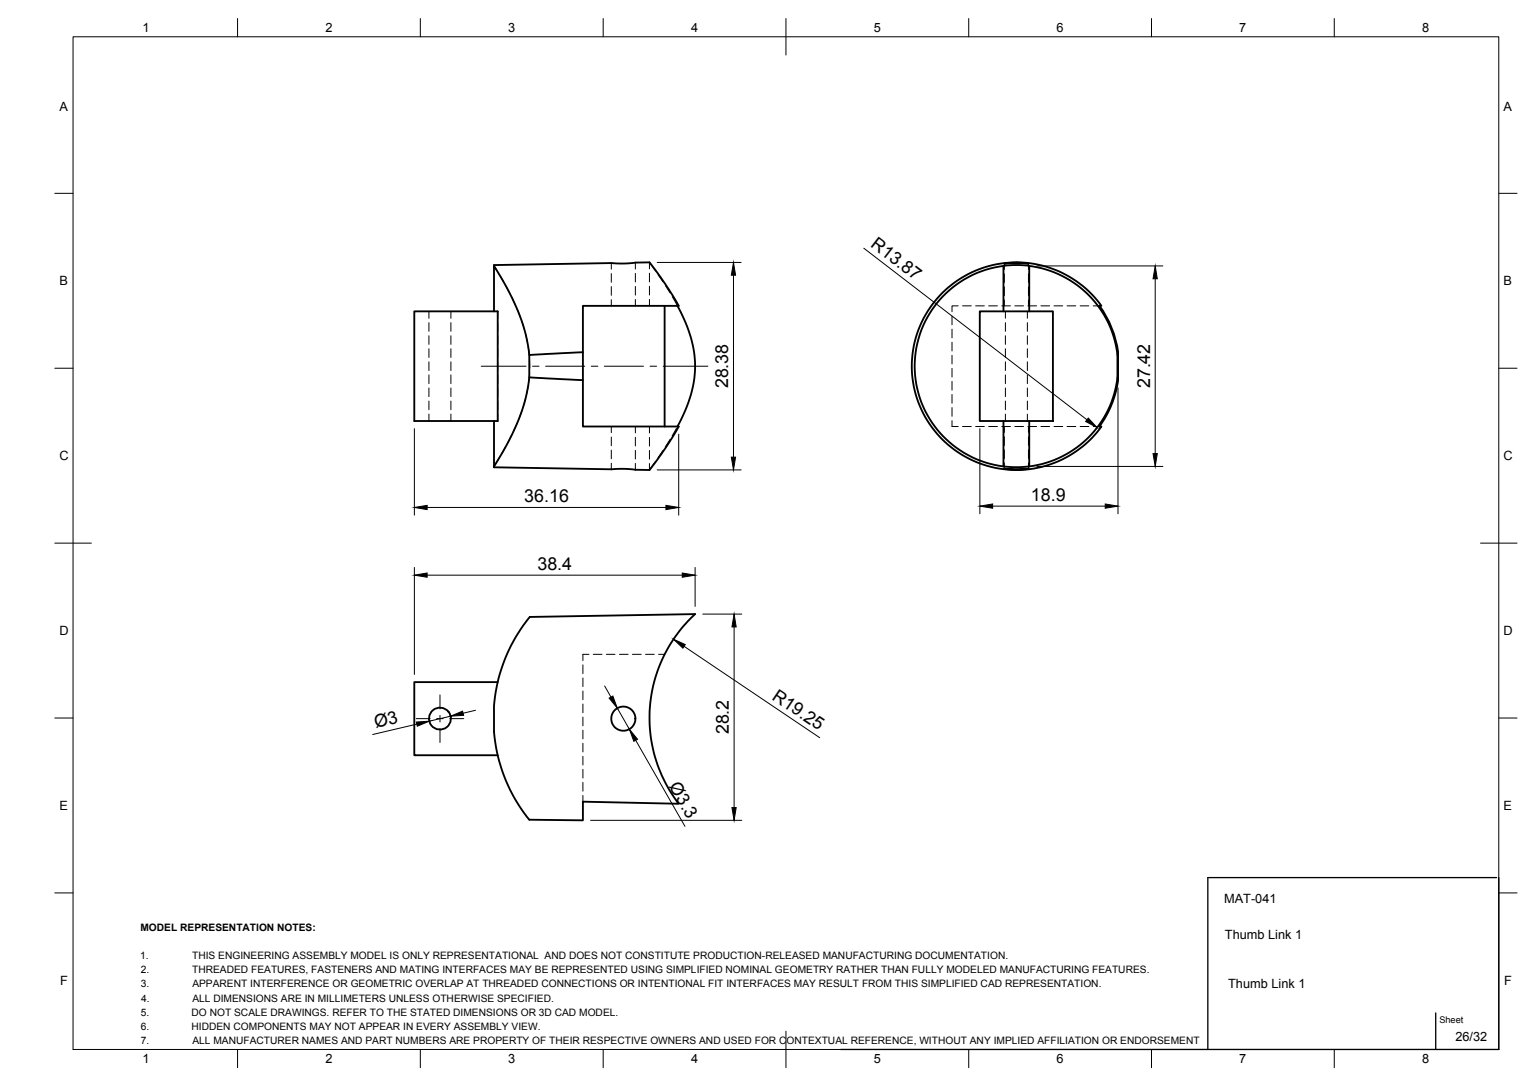
ISO-10303-21;
HEADER;
/* Generated by software containing ST-Developer
 * from STEP Tools, Inc. (www.steptools.com) 
 */

FILE_DESCRIPTION(
/* description */ ('STEP AP214'),
/* implementation_level */ '2;1');

FILE_NAME(
/* name */ 'Thumb Link 1.step',
/* time_stamp */ '2026-11-14T21:57:47-08:00',
/* author */ (''),
/* organization */ (''),
/* preprocessor_version */ 'ST-DEVELOPER v20.2',
/* originating_system */ 'Autodesk Translation Framework v15.17.0.0',
/* authorisation */ '');

FILE_SCHEMA (('AUTOMOTIVE_DESIGN { 1 0 10303 214 3 1 1 }'));
ENDSEC;

DATA;
#10=MECHANICAL_DESIGN_GEOMETRIC_PRESENTATION_REPRESENTATION('',(#261),#13199);
#12=(
BOUNDED_CURVE()
B_SPLINE_CURVE(2,(#12481,#12482,#12483),.UNSPECIFIED.,.F.,.F.)
B_SPLINE_CURVE_WITH_KNOTS((3,3),(-1.60124615225297,-0.808783730274253),
 .UNSPECIFIED.)
CURVE()
GEOMETRIC_REPRESENTATION_ITEM()
RATIONAL_B_SPLINE_CURVE((1.00284139361103,1.00297035013721,1.00227572336188))
REPRESENTATION_ITEM('')
);
#13=(
BOUNDED_CURVE()
B_SPLINE_CURVE(2,(#12547,#12548,#12549),.UNSPECIFIED.,.F.,.F.)
B_SPLINE_CURVE_WITH_KNOTS((3,3),(-2.14592066681242,-1.35342729440919),
 .UNSPECIFIED.)
CURVE()
GEOMETRIC_REPRESENTATION_ITEM()
RATIONAL_B_SPLINE_CURVE((1.00227603694351,1.00297081766941,1.00284201479666))
REPRESENTATION_ITEM('')
);
#123=CONICAL_SURFACE('',#7682,14.3,0.0174532925199433);
#189=B_SPLINE_CURVE_WITH_KNOTS('',3,(#12314,#12315,#12316,#12317,#12318,
#12319,#12320,#12321,#12322,#12323,#12324,#12325,#12326,#12327,#12328,#12329,
#12330,#12331),.UNSPECIFIED.,.F.,.F.,(4,2,2,2,2,2,2,2,4),(1.2439344005176,
1.30605868780294,1.36818297508828,1.43027366468746,1.49236435428665,1.55470347254014,
1.61704259079363,1.67936460734276,1.74168662389188),.UNSPECIFIED.);
#190=B_SPLINE_CURVE_WITH_KNOTS('',3,(#12332,#12333,#12334,#12335,#12336,
#12337,#12338,#12339,#12340,#12341,#12342,#12343,#12344,#12345,#12346,#12347,
#12348,#12349,#12350),.UNSPECIFIED.,.F.,.F.,(4,2,2,2,3,2,2,2,4),(0.746182177143323,
0.80850419369245,0.870826210241576,0.933165328495069,0.995504446748561,
1.05759513634774,1.11968582594693,1.18181011323227,1.2439344005176),
 .UNSPECIFIED.);
#191=B_SPLINE_CURVE_WITH_KNOTS('',3,(#12354,#12355,#12356,#12357,#12358,
#12359,#12360,#12361,#12362,#12363,#12364,#12365,#12366,#12367,#12368,#12369,
#12370,#12371),.UNSPECIFIED.,.F.,.F.,(4,2,2,2,2,2,2,2,4),(-0.746182177143323,
-0.683860160594197,-0.621538144045071,-0.559199025791578,-0.496859907538086,
-0.434769217938902,-0.372678528339718,-0.310554241054381,-0.248429953769043),
 .UNSPECIFIED.);
#192=B_SPLINE_CURVE_WITH_KNOTS('',3,(#12375,#12376,#12377,#12378,#12379,
#12380,#12381,#12382,#12383,#12384,#12385,#12386,#12387,#12388,#12389,#12390,
#12391,#12392,#12393),.UNSPECIFIED.,.F.,.F.,(4,2,2,2,3,2,2,2,4),(-0.248429953769043,
-0.186305666483705,-0.124181379198368,-0.0620906895991839,0.,0.0623391182534924,
0.124678236506985,0.187000253056111,0.249322269605238),.UNSPECIFIED.);
#193=B_SPLINE_CURVE_WITH_KNOTS('',3,(#12409,#12410,#12411,#12412,#12413,
#12414,#12415,#12416,#12417,#12418,#12419,#12420,#12421,#12422),
 .UNSPECIFIED.,.F.,.F.,(4,2,2,2,2,2,4),(6.66820605648738,6.76341848404012,
7.03258976532484,7.57093232789428,8.11497235847169,8.3869923737604,8.50692180294266),
 .UNSPECIFIED.);
#194=B_SPLINE_CURVE_WITH_KNOTS('',3,(#12426,#12427,#12428,#12429,#12430,
#12431,#12432,#12433,#12434,#12435,#12436,#12437,#12438,#12439),
 .UNSPECIFIED.,.F.,.F.,(4,2,2,2,2,2,4),(0.152090586106455,0.272020015288707,
0.544040030577415,1.08808006115483,1.62642262372427,1.89559390500899,1.99080633256173),
 .UNSPECIFIED.);
#195=B_SPLINE_CURVE_WITH_KNOTS('',3,(#12452,#12453,#12454,#12455,#12456,
#12457,#12458,#12459,#12460,#12461,#12462,#12463,#12464,#12465,#12466,#12467,
#12468,#12469,#12470,#12471,#12472,#12473,#12474,#12475,#12476,#12477),
 .UNSPECIFIED.,.F.,.F.,(4,2,2,2,2,2,2,2,2,2,2,2,4),(2.33883536058546,2.43393235013178,
2.70309951396985,3.24143384164599,3.78547001808527,4.05748810630491,4.32950619452455,
4.6015242827442,4.87354237096384,5.41757854740312,5.95591287507926,6.22508003891732,
6.32017702846365),.UNSPECIFIED.);
#196=B_SPLINE_CURVE_WITH_KNOTS('',3,(#12487,#12488,#12489,#12490,#12491,
#12492,#12493),.UNSPECIFIED.,.F.,.F.,(4,3,4),(0.0272601210138638,0.0280070000945348,
0.0403698029815644),.UNSPECIFIED.);
#197=B_SPLINE_CURVE_WITH_KNOTS('',3,(#12495,#12496,#12497,#12498,#12499,
#12500,#12501,#12502,#12503,#12504,#12505,#12506,#12507,#12508,#12509,#12510,
#12511,#12512,#12513,#12514,#12515,#12516,#12517,#12518,#12519,#12520,#12521,
#12522,#12523,#12524,#12525,#12526,#12527,#12528,#12529,#12530,#12531,#12532,
#12533,#12534,#12535,#12536),.UNSPECIFIED.,.F.,.F.,(4,2,2,2,2,2,2,2,2,2,
2,2,2,2,2,2,2,2,2,2,4),(0.895792364322182,1.15266269025927,1.7130326392156,
1.99321761369377,2.27340258817193,2.55312809524007,2.8328536023082,3.39230461644446,
3.9653006408784,4.25179865309537,4.53829666531233,4.8247946775293,5.11129268974627,
5.6842887141802,6.24373972831647,6.5234652353846,6.80319074245273,7.08415066001029,
7.36511057756785,7.92703041268297,8.1809357022053),.UNSPECIFIED.);
#198=B_SPLINE_CURVE_WITH_KNOTS('',3,(#12538,#12539,#12540,#12541,#12542,
#12543,#12544),.UNSPECIFIED.,.F.,.F.,(4,3,4),(0.01564419735118,0.0280070001942108,
0.0287538792722237),.UNSPECIFIED.);
#225=SHAPE_REPRESENTATION_RELATIONSHIP('SRR','None',#13297,#243);
#243=ADVANCED_BREP_SHAPE_REPRESENTATION('',(#279),#13193);
#261=STYLED_ITEM('',(#13411),#279);
#279=MANIFOLD_SOLID_BREP('Body1',#6856);
#362=FACE_BOUND('',#2584,.T.);
#363=FACE_BOUND('',#2585,.T.);
#364=FACE_BOUND('',#2590,.T.);
#365=FACE_BOUND('',#2592,.T.);
#366=FACE_BOUND('',#2599,.T.);
#367=FACE_BOUND('',#2601,.T.);
#561=PLANE('',#7674);
#562=PLANE('',#7686);
#563=PLANE('',#7687);
#564=PLANE('',#7691);
#565=PLANE('',#7692);
#566=PLANE('',#7693);
#567=PLANE('',#7694);
#568=PLANE('',#7695);
#569=PLANE('',#7696);
#570=PLANE('',#7697);
#571=PLANE('',#7698);
#572=PLANE('',#7699);
#1017=LINE('',#12306,#1535);
#1018=LINE('',#12312,#1536);
#1019=LINE('',#12373,#1537);
#1020=LINE('',#12397,#1538);
#1021=LINE('',#12399,#1539);
#1022=LINE('',#12401,#1540);
#1023=LINE('',#12406,#1541);
#1024=LINE('',#12424,#1542);
#1025=LINE('',#12441,#1543);
#1026=LINE('',#12447,#1544);
#1027=LINE('',#12451,#1545);
#1028=LINE('',#12551,#1546);
#1029=LINE('',#12553,#1547);
#1030=LINE('',#12557,#1548);
#1031=LINE('',#12562,#1549);
#1032=LINE('',#12563,#1550);
#1033=LINE('',#12566,#1551);
#1034=LINE('',#12567,#1552);
#1035=LINE('',#12569,#1553);
#1036=LINE('',#12573,#1554);
#1037=LINE('',#12575,#1555);
#1038=LINE('',#12576,#1556);
#1039=LINE('',#12579,#1557);
#1040=LINE('',#12581,#1558);
#1041=LINE('',#12582,#1559);
#1042=LINE('',#12584,#1560);
#1043=LINE('',#12585,#1561);
#1535=VECTOR('',#9454,1.5);
#1536=VECTOR('',#9461,1.65);
#1537=VECTOR('',#9464,1.65);
#1538=VECTOR('',#9469,1000.);
#1539=VECTOR('',#9470,1000.);
#1540=VECTOR('',#9471,1000.);
#1541=VECTOR('',#9476,1000.);
#1542=VECTOR('',#9479,1000.);
#1543=VECTOR('',#9480,1000.);
#1544=VECTOR('',#9487,1000.);
#1545=VECTOR('',#9490,1000.);
#1546=VECTOR('',#9501,1000.);
#1547=VECTOR('',#9504,1000.);
#1548=VECTOR('',#9507,1000.);
#1549=VECTOR('',#9514,1000.);
#1550=VECTOR('',#9515,1000.);
#1551=VECTOR('',#9518,1000.);
#1552=VECTOR('',#9519,1000.);
#1553=VECTOR('',#9522,1000.);
#1554=VECTOR('',#9527,1000.);
#1555=VECTOR('',#9528,1000.);
#1556=VECTOR('',#9529,1000.);
#1557=VECTOR('',#9532,1000.);
#1558=VECTOR('',#9533,1000.);
#1559=VECTOR('',#9534,1000.);
#1560=VECTOR('',#9537,1000.);
#1561=VECTOR('',#9538,1000.);
#1761=CYLINDRICAL_SURFACE('',#7667,1.5);
#1762=CYLINDRICAL_SURFACE('',#7670,1.65);
#1763=CYLINDRICAL_SURFACE('',#7672,1.65);
#1764=CYLINDRICAL_SURFACE('',#7676,21.9689920245294);
#1765=CYLINDRICAL_SURFACE('',#7679,21.9689920245294);
#1766=CYLINDRICAL_SURFACE('',#7688,19.25);
#2108=FACE_OUTER_BOUND('',#2577,.T.);
#2109=FACE_OUTER_BOUND('',#2578,.T.);
#2110=FACE_OUTER_BOUND('',#2579,.T.);
#2111=FACE_OUTER_BOUND('',#2580,.T.);
#2112=FACE_OUTER_BOUND('',#2581,.T.);
#2113=FACE_OUTER_BOUND('',#2582,.T.);
#2114=FACE_OUTER_BOUND('',#2583,.T.);
#2115=FACE_OUTER_BOUND('',#2586,.T.);
#2116=FACE_OUTER_BOUND('',#2587,.T.);
#2117=FACE_OUTER_BOUND('',#2588,.T.);
#2118=FACE_OUTER_BOUND('',#2589,.T.);
#2119=FACE_OUTER_BOUND('',#2591,.T.);
#2120=FACE_OUTER_BOUND('',#2593,.T.);
#2121=FACE_OUTER_BOUND('',#2594,.T.);
#2122=FACE_OUTER_BOUND('',#2595,.T.);
#2123=FACE_OUTER_BOUND('',#2596,.T.);
#2124=FACE_OUTER_BOUND('',#2597,.T.);
#2125=FACE_OUTER_BOUND('',#2598,.T.);
#2126=FACE_OUTER_BOUND('',#2600,.T.);
#2577=EDGE_LOOP('',(#6032,#6033,#6034,#6035));
#2578=EDGE_LOOP('',(#6036,#6037,#6038,#6039,#6040));
#2579=EDGE_LOOP('',(#6041,#6042,#6043,#6044,#6045));
#2580=EDGE_LOOP('',(#6046,#6047,#6048,#6049));
#2581=EDGE_LOOP('',(#6050,#6051,#6052,#6053,#6054,#6055,#6056,#6057));
#2582=EDGE_LOOP('',(#6058,#6059,#6060,#6061,#6062,#6063));
#2583=EDGE_LOOP('',(#6064,#6065,#6066,#6067,#6068,#6069,#6070,#6071,#6072,
#6073,#6074,#6075));
#2584=EDGE_LOOP('',(#6076,#6077));
#2585=EDGE_LOOP('',(#6078,#6079));
#2586=EDGE_LOOP('',(#6080,#6081,#6082,#6083));
#2587=EDGE_LOOP('',(#6084,#6085,#6086,#6087));
#2588=EDGE_LOOP('',(#6088,#6089,#6090,#6091));
#2589=EDGE_LOOP('',(#6092,#6093,#6094,#6095));
#2590=EDGE_LOOP('',(#6096));
#2591=EDGE_LOOP('',(#6097,#6098,#6099,#6100));
#2592=EDGE_LOOP('',(#6101));
#2593=EDGE_LOOP('',(#6102,#6103,#6104,#6105,#6106,#6107));
#2594=EDGE_LOOP('',(#6108,#6109,#6110,#6111));
#2595=EDGE_LOOP('',(#6112,#6113,#6114,#6115));
#2596=EDGE_LOOP('',(#6116,#6117,#6118,#6119));
#2597=EDGE_LOOP('',(#6120,#6121,#6122,#6123));
#2598=EDGE_LOOP('',(#6124,#6125,#6126,#6127,#6128,#6129));
#2599=EDGE_LOOP('',(#6130));
#2600=EDGE_LOOP('',(#6131,#6132,#6133,#6134,#6135,#6136));
#2601=EDGE_LOOP('',(#6137));
#2939=CIRCLE('',#7668,1.5);
#2940=CIRCLE('',#7669,1.5);
#2941=CIRCLE('',#7671,1.65);
#2942=CIRCLE('',#7673,1.65);
#2943=CIRCLE('',#7675,13.819985714474);
#2944=CIRCLE('',#7677,21.9689920245294);
#2945=CIRCLE('',#7678,21.9689920245294);
#2946=CIRCLE('',#7680,21.9689920245294);
#2947=CIRCLE('',#7681,21.9689920245294);
#2948=CIRCLE('',#7683,13.819985714474);
#2949=CIRCLE('',#7684,14.0321508983363);
#2950=CIRCLE('',#7685,14.0321508983363);
#2951=CIRCLE('',#7689,19.25);
#2952=CIRCLE('',#7690,19.25);
#3479=VERTEX_POINT('',#12303);
#3480=VERTEX_POINT('',#12305);
#3481=VERTEX_POINT('',#12309);
#3482=VERTEX_POINT('',#12311);
#3483=VERTEX_POINT('',#12313);
#3484=VERTEX_POINT('',#12352);
#3485=VERTEX_POINT('',#12353);
#3486=VERTEX_POINT('',#12372);
#3487=VERTEX_POINT('',#12395);
#3488=VERTEX_POINT('',#12396);
#3489=VERTEX_POINT('',#12398);
#3490=VERTEX_POINT('',#12400);
#3491=VERTEX_POINT('',#12404);
#3492=VERTEX_POINT('',#12405);
#3493=VERTEX_POINT('',#12408);
#3494=VERTEX_POINT('',#12423);
#3495=VERTEX_POINT('',#12425);
#3496=VERTEX_POINT('',#12440);
#3497=VERTEX_POINT('',#12444);
#3498=VERTEX_POINT('',#12446);
#3499=VERTEX_POINT('',#12448);
#3500=VERTEX_POINT('',#12450);
#3501=VERTEX_POINT('',#12480);
#3502=VERTEX_POINT('',#12484);
#3503=VERTEX_POINT('',#12486);
#3504=VERTEX_POINT('',#12494);
#3505=VERTEX_POINT('',#12537);
#3506=VERTEX_POINT('',#12545);
#3507=VERTEX_POINT('',#12555);
#3508=VERTEX_POINT('',#12556);
#3509=VERTEX_POINT('',#12561);
#3510=VERTEX_POINT('',#12565);
#3511=VERTEX_POINT('',#12572);
#3512=VERTEX_POINT('',#12574);
#3513=VERTEX_POINT('',#12578);
#3514=VERTEX_POINT('',#12580);
#4353=EDGE_CURVE('',#3479,#3479,#2939,.T.);
#4354=EDGE_CURVE('',#3479,#3480,#1017,.T.);
#4355=EDGE_CURVE('',#3480,#3480,#2940,.T.);
#4356=EDGE_CURVE('',#3481,#3481,#2941,.T.);
#4357=EDGE_CURVE('',#3481,#3482,#1018,.T.);
#4358=EDGE_CURVE('',#3482,#3483,#189,.T.);
#4359=EDGE_CURVE('',#3483,#3482,#190,.T.);
#4360=EDGE_CURVE('',#3484,#3485,#191,.T.);
#4361=EDGE_CURVE('',#3485,#3486,#1019,.T.);
#4362=EDGE_CURVE('',#3486,#3486,#2942,.T.);
#4363=EDGE_CURVE('',#3485,#3484,#192,.T.);
#4364=EDGE_CURVE('',#3487,#3488,#1020,.T.);
#4365=EDGE_CURVE('',#3488,#3489,#1021,.T.);
#4366=EDGE_CURVE('',#3489,#3490,#1022,.T.);
#4367=EDGE_CURVE('',#3490,#3487,#2943,.T.);
#4368=EDGE_CURVE('',#3491,#3492,#1023,.T.);
#4369=EDGE_CURVE('',#3491,#3488,#2944,.T.);
#4370=EDGE_CURVE('',#3487,#3493,#193,.T.);
#4371=EDGE_CURVE('',#3494,#3493,#1024,.T.);
#4372=EDGE_CURVE('',#3494,#3495,#194,.T.);
#4373=EDGE_CURVE('',#3496,#3495,#1025,.T.);
#4374=EDGE_CURVE('',#3492,#3496,#2945,.T.);
#4375=EDGE_CURVE('',#3489,#3497,#2946,.T.);
#4376=EDGE_CURVE('',#3498,#3497,#1026,.T.);
#4377=EDGE_CURVE('',#3499,#3498,#2947,.T.);
#4378=EDGE_CURVE('',#3500,#3499,#1027,.T.);
#4379=EDGE_CURVE('',#3500,#3490,#195,.T.);
#4380=EDGE_CURVE('',#3495,#3500,#2948,.T.);
#4381=EDGE_CURVE('',#3501,#3494,#12,.T.);
#4382=EDGE_CURVE('',#3502,#3501,#2949,.T.);
#4383=EDGE_CURVE('',#3503,#3502,#196,.T.);
#4384=EDGE_CURVE('',#3504,#3503,#197,.T.);
#4385=EDGE_CURVE('',#3505,#3504,#198,.T.);
#4386=EDGE_CURVE('',#3506,#3505,#2950,.T.);
#4387=EDGE_CURVE('',#3493,#3506,#13,.T.);
#4388=EDGE_CURVE('',#3506,#3501,#1028,.T.);
#4389=EDGE_CURVE('',#3496,#3499,#1029,.T.);
#4390=EDGE_CURVE('',#3507,#3508,#1030,.T.);
#4391=EDGE_CURVE('',#3507,#3504,#2951,.T.);
#4392=EDGE_CURVE('',#3503,#3508,#2952,.T.);
#4393=EDGE_CURVE('',#3509,#3507,#1031,.T.);
#4394=EDGE_CURVE('',#3505,#3509,#1032,.T.);
#4395=EDGE_CURVE('',#3502,#3510,#1033,.T.);
#4396=EDGE_CURVE('',#3508,#3510,#1034,.T.);
#4397=EDGE_CURVE('',#3510,#3509,#1035,.T.);
#4398=EDGE_CURVE('',#3511,#3491,#1036,.T.);
#4399=EDGE_CURVE('',#3512,#3492,#1037,.T.);
#4400=EDGE_CURVE('',#3511,#3512,#1038,.T.);
#4401=EDGE_CURVE('',#3513,#3512,#1039,.T.);
#4402=EDGE_CURVE('',#3514,#3513,#1040,.T.);
#4403=EDGE_CURVE('',#3514,#3511,#1041,.T.);
#4404=EDGE_CURVE('',#3498,#3513,#1042,.T.);
#4405=EDGE_CURVE('',#3497,#3514,#1043,.T.);
#6032=ORIENTED_EDGE('',*,*,#4353,.F.);
#6033=ORIENTED_EDGE('',*,*,#4354,.T.);
#6034=ORIENTED_EDGE('',*,*,#4355,.T.);
#6035=ORIENTED_EDGE('',*,*,#4354,.F.);
#6036=ORIENTED_EDGE('',*,*,#4356,.F.);
#6037=ORIENTED_EDGE('',*,*,#4357,.T.);
#6038=ORIENTED_EDGE('',*,*,#4358,.T.);
#6039=ORIENTED_EDGE('',*,*,#4359,.T.);
#6040=ORIENTED_EDGE('',*,*,#4357,.F.);
#6041=ORIENTED_EDGE('',*,*,#4360,.T.);
#6042=ORIENTED_EDGE('',*,*,#4361,.T.);
#6043=ORIENTED_EDGE('',*,*,#4362,.F.);
#6044=ORIENTED_EDGE('',*,*,#4361,.F.);
#6045=ORIENTED_EDGE('',*,*,#4363,.T.);
#6046=ORIENTED_EDGE('',*,*,#4364,.T.);
#6047=ORIENTED_EDGE('',*,*,#4365,.T.);
#6048=ORIENTED_EDGE('',*,*,#4366,.T.);
#6049=ORIENTED_EDGE('',*,*,#4367,.T.);
#6050=ORIENTED_EDGE('',*,*,#4368,.F.);
#6051=ORIENTED_EDGE('',*,*,#4369,.T.);
#6052=ORIENTED_EDGE('',*,*,#4364,.F.);
#6053=ORIENTED_EDGE('',*,*,#4370,.T.);
#6054=ORIENTED_EDGE('',*,*,#4371,.F.);
#6055=ORIENTED_EDGE('',*,*,#4372,.T.);
#6056=ORIENTED_EDGE('',*,*,#4373,.F.);
#6057=ORIENTED_EDGE('',*,*,#4374,.F.);
#6058=ORIENTED_EDGE('',*,*,#4366,.F.);
#6059=ORIENTED_EDGE('',*,*,#4375,.T.);
#6060=ORIENTED_EDGE('',*,*,#4376,.F.);
#6061=ORIENTED_EDGE('',*,*,#4377,.F.);
#6062=ORIENTED_EDGE('',*,*,#4378,.F.);
#6063=ORIENTED_EDGE('',*,*,#4379,.T.);
#6064=ORIENTED_EDGE('',*,*,#4379,.F.);
#6065=ORIENTED_EDGE('',*,*,#4380,.F.);
#6066=ORIENTED_EDGE('',*,*,#4372,.F.);
#6067=ORIENTED_EDGE('',*,*,#4381,.F.);
#6068=ORIENTED_EDGE('',*,*,#4382,.F.);
#6069=ORIENTED_EDGE('',*,*,#4383,.F.);
#6070=ORIENTED_EDGE('',*,*,#4384,.F.);
#6071=ORIENTED_EDGE('',*,*,#4385,.F.);
#6072=ORIENTED_EDGE('',*,*,#4386,.F.);
#6073=ORIENTED_EDGE('',*,*,#4387,.F.);
#6074=ORIENTED_EDGE('',*,*,#4370,.F.);
#6075=ORIENTED_EDGE('',*,*,#4367,.F.);
#6076=ORIENTED_EDGE('',*,*,#4359,.F.);
#6077=ORIENTED_EDGE('',*,*,#4358,.F.);
#6078=ORIENTED_EDGE('',*,*,#4360,.F.);
#6079=ORIENTED_EDGE('',*,*,#4363,.F.);
#6080=ORIENTED_EDGE('',*,*,#4381,.T.);
#6081=ORIENTED_EDGE('',*,*,#4371,.T.);
#6082=ORIENTED_EDGE('',*,*,#4387,.T.);
#6083=ORIENTED_EDGE('',*,*,#4388,.T.);
#6084=ORIENTED_EDGE('',*,*,#4389,.F.);
#6085=ORIENTED_EDGE('',*,*,#4373,.T.);
#6086=ORIENTED_EDGE('',*,*,#4380,.T.);
#6087=ORIENTED_EDGE('',*,*,#4378,.T.);
#6088=ORIENTED_EDGE('',*,*,#4390,.F.);
#6089=ORIENTED_EDGE('',*,*,#4391,.T.);
#6090=ORIENTED_EDGE('',*,*,#4384,.T.);
#6091=ORIENTED_EDGE('',*,*,#4392,.T.);
#6092=ORIENTED_EDGE('',*,*,#4385,.T.);
#6093=ORIENTED_EDGE('',*,*,#4391,.F.);
#6094=ORIENTED_EDGE('',*,*,#4393,.F.);
#6095=ORIENTED_EDGE('',*,*,#4394,.F.);
#6096=ORIENTED_EDGE('',*,*,#4356,.T.);
#6097=ORIENTED_EDGE('',*,*,#4383,.T.);
#6098=ORIENTED_EDGE('',*,*,#4395,.T.);
#6099=ORIENTED_EDGE('',*,*,#4396,.F.);
#6100=ORIENTED_EDGE('',*,*,#4392,.F.);
#6101=ORIENTED_EDGE('',*,*,#4362,.T.);
#6102=ORIENTED_EDGE('',*,*,#4382,.T.);
#6103=ORIENTED_EDGE('',*,*,#4388,.F.);
#6104=ORIENTED_EDGE('',*,*,#4386,.T.);
#6105=ORIENTED_EDGE('',*,*,#4394,.T.);
#6106=ORIENTED_EDGE('',*,*,#4397,.F.);
#6107=ORIENTED_EDGE('',*,*,#4395,.F.);
#6108=ORIENTED_EDGE('',*,*,#4390,.T.);
#6109=ORIENTED_EDGE('',*,*,#4396,.T.);
#6110=ORIENTED_EDGE('',*,*,#4397,.T.);
#6111=ORIENTED_EDGE('',*,*,#4393,.T.);
#6112=ORIENTED_EDGE('',*,*,#4398,.T.);
#6113=ORIENTED_EDGE('',*,*,#4368,.T.);
#6114=ORIENTED_EDGE('',*,*,#4399,.F.);
#6115=ORIENTED_EDGE('',*,*,#4400,.F.);
#6116=ORIENTED_EDGE('',*,*,#4400,.T.);
#6117=ORIENTED_EDGE('',*,*,#4401,.F.);
#6118=ORIENTED_EDGE('',*,*,#4402,.F.);
#6119=ORIENTED_EDGE('',*,*,#4403,.T.);
#6120=ORIENTED_EDGE('',*,*,#4404,.F.);
#6121=ORIENTED_EDGE('',*,*,#4376,.T.);
#6122=ORIENTED_EDGE('',*,*,#4405,.T.);
#6123=ORIENTED_EDGE('',*,*,#4402,.T.);
#6124=ORIENTED_EDGE('',*,*,#4369,.F.);
#6125=ORIENTED_EDGE('',*,*,#4398,.F.);
#6126=ORIENTED_EDGE('',*,*,#4403,.F.);
#6127=ORIENTED_EDGE('',*,*,#4405,.F.);
#6128=ORIENTED_EDGE('',*,*,#4375,.F.);
#6129=ORIENTED_EDGE('',*,*,#4365,.F.);
#6130=ORIENTED_EDGE('',*,*,#4353,.T.);
#6131=ORIENTED_EDGE('',*,*,#4399,.T.);
#6132=ORIENTED_EDGE('',*,*,#4374,.T.);
#6133=ORIENTED_EDGE('',*,*,#4389,.T.);
#6134=ORIENTED_EDGE('',*,*,#4377,.T.);
#6135=ORIENTED_EDGE('',*,*,#4404,.T.);
#6136=ORIENTED_EDGE('',*,*,#4401,.T.);
#6137=ORIENTED_EDGE('',*,*,#4355,.F.);
#6760=ADVANCED_FACE('',(#2108),#1761,.F.);
#6761=ADVANCED_FACE('',(#2109),#1762,.F.);
#6762=ADVANCED_FACE('',(#2110),#1763,.F.);
#6763=ADVANCED_FACE('',(#2111),#561,.T.);
#6764=ADVANCED_FACE('',(#2112),#1764,.T.);
#6765=ADVANCED_FACE('',(#2113),#1765,.T.);
#6766=ADVANCED_FACE('',(#2114,#362,#363),#123,.T.);
#6767=ADVANCED_FACE('',(#2115),#562,.T.);
#6768=ADVANCED_FACE('',(#2116),#563,.T.);
#6769=ADVANCED_FACE('',(#2117),#1766,.F.);
#6770=ADVANCED_FACE('',(#2118,#364),#564,.T.);
#6771=ADVANCED_FACE('',(#2119,#365),#565,.T.);
#6772=ADVANCED_FACE('',(#2120),#566,.T.);
#6773=ADVANCED_FACE('',(#2121),#567,.F.);
#6774=ADVANCED_FACE('',(#2122),#568,.T.);
#6775=ADVANCED_FACE('',(#2123),#569,.T.);
#6776=ADVANCED_FACE('',(#2124),#570,.T.);
#6777=ADVANCED_FACE('',(#2125,#366),#571,.F.);
#6778=ADVANCED_FACE('',(#2126,#367),#572,.T.);
#6856=CLOSED_SHELL('',(#6760,#6761,#6762,#6763,#6764,#6765,#6766,#6767,
#6768,#6769,#6770,#6771,#6772,#6773,#6774,#6775,#6776,#6777,#6778));
#7666=AXIS2_PLACEMENT_3D('',#12301,#9448,#9449);
#7667=AXIS2_PLACEMENT_3D('',#12302,#9450,#9451);
#7668=AXIS2_PLACEMENT_3D('',#12304,#9452,#9453);
#7669=AXIS2_PLACEMENT_3D('',#12307,#9455,#9456);
#7670=AXIS2_PLACEMENT_3D('',#12308,#9457,#9458);
#7671=AXIS2_PLACEMENT_3D('',#12310,#9459,#9460);
#7672=AXIS2_PLACEMENT_3D('',#12351,#9462,#9463);
#7673=AXIS2_PLACEMENT_3D('',#12374,#9465,#9466);
#7674=AXIS2_PLACEMENT_3D('',#12394,#9467,#9468);
#7675=AXIS2_PLACEMENT_3D('',#12402,#9472,#9473);
#7676=AXIS2_PLACEMENT_3D('',#12403,#9474,#9475);
#7677=AXIS2_PLACEMENT_3D('',#12407,#9477,#9478);
#7678=AXIS2_PLACEMENT_3D('',#12442,#9481,#9482);
#7679=AXIS2_PLACEMENT_3D('',#12443,#9483,#9484);
#7680=AXIS2_PLACEMENT_3D('',#12445,#9485,#9486);
#7681=AXIS2_PLACEMENT_3D('',#12449,#9488,#9489);
#7682=AXIS2_PLACEMENT_3D('',#12478,#9491,#9492);
#7683=AXIS2_PLACEMENT_3D('',#12479,#9493,#9494);
#7684=AXIS2_PLACEMENT_3D('',#12485,#9495,#9496);
#7685=AXIS2_PLACEMENT_3D('',#12546,#9497,#9498);
#7686=AXIS2_PLACEMENT_3D('',#12550,#9499,#9500);
#7687=AXIS2_PLACEMENT_3D('',#12552,#9502,#9503);
#7688=AXIS2_PLACEMENT_3D('',#12554,#9505,#9506);
#7689=AXIS2_PLACEMENT_3D('',#12558,#9508,#9509);
#7690=AXIS2_PLACEMENT_3D('',#12559,#9510,#9511);
#7691=AXIS2_PLACEMENT_3D('',#12560,#9512,#9513);
#7692=AXIS2_PLACEMENT_3D('',#12564,#9516,#9517);
#7693=AXIS2_PLACEMENT_3D('',#12568,#9520,#9521);
#7694=AXIS2_PLACEMENT_3D('',#12570,#9523,#9524);
#7695=AXIS2_PLACEMENT_3D('',#12571,#9525,#9526);
#7696=AXIS2_PLACEMENT_3D('',#12577,#9530,#9531);
#7697=AXIS2_PLACEMENT_3D('',#12583,#9535,#9536);
#7698=AXIS2_PLACEMENT_3D('',#12586,#9539,#9540);
#7699=AXIS2_PLACEMENT_3D('',#12587,#9541,#9542);
#9448=DIRECTION('axis',(0.,0.,1.));
#9449=DIRECTION('refdir',(1.,0.,0.));
#9450=DIRECTION('center_axis',(0.,1.,0.));
#9451=DIRECTION('ref_axis',(0.,0.,1.));
#9452=DIRECTION('center_axis',(0.,1.,0.));
#9453=DIRECTION('ref_axis',(0.,0.,1.));
#9454=DIRECTION('',(0.,1.,0.));
#9455=DIRECTION('center_axis',(0.,1.,0.));
#9456=DIRECTION('ref_axis',(0.,0.,1.));
#9457=DIRECTION('center_axis',(0.,-1.,0.));
#9458=DIRECTION('ref_axis',(0.,0.,-1.));
#9459=DIRECTION('center_axis',(0.,-1.,-1.24352412568707E-16));
#9460=DIRECTION('ref_axis',(0.,-1.24352412568707E-16,1.));
#9461=DIRECTION('',(0.,-1.,0.));
#9462=DIRECTION('center_axis',(0.,-1.,0.));
#9463=DIRECTION('ref_axis',(0.,0.,-1.));
#9464=DIRECTION('',(0.,-1.,0.));
#9465=DIRECTION('center_axis',(0.,1.,1.24352412568707E-16));
#9466=DIRECTION('ref_axis',(0.,1.24352412568707E-16,-1.));
#9467=DIRECTION('center_axis',(0.,0.,1.));
#9468=DIRECTION('ref_axis',(1.,0.,0.));
#9469=DIRECTION('',(0.,1.,0.));
#9470=DIRECTION('',(-1.,0.,0.));
#9471=DIRECTION('',(0.,-1.,0.));
#9472=DIRECTION('center_axis',(0.,0.,1.));
#9473=DIRECTION('ref_axis',(1.,0.,0.));
#9474=DIRECTION('center_axis',(0.,-1.,0.));
#9475=DIRECTION('ref_axis',(0.,0.,-1.));
#9476=DIRECTION('',(0.,1.,0.));
#9477=DIRECTION('center_axis',(0.,-1.,0.));
#9478=DIRECTION('ref_axis',(-4.44101590494474E-15,0.,1.));
#9479=DIRECTION('',(0.,-1.,0.));
#9480=DIRECTION('',(0.,1.,0.));
#9481=DIRECTION('center_axis',(0.,-1.,0.));
#9482=DIRECTION('ref_axis',(-4.44101590494474E-15,0.,1.));
#9483=DIRECTION('center_axis',(0.,-1.,0.));
#9484=DIRECTION('ref_axis',(0.,0.,-1.));
#9485=DIRECTION('center_axis',(0.,-1.,0.));
#9486=DIRECTION('ref_axis',(0.,0.,1.));
#9487=DIRECTION('',(0.,-1.,0.));
#9488=DIRECTION('center_axis',(0.,-1.,0.));
#9489=DIRECTION('ref_axis',(0.,0.,1.));
#9490=DIRECTION('',(0.,-1.,0.));
#9491=DIRECTION('center_axis',(0.,0.,-1.));
#9492=DIRECTION('ref_axis',(-1.,-1.22464679914735E-16,0.));
#9493=DIRECTION('center_axis',(0.,0.,1.));
#9494=DIRECTION('ref_axis',(1.,0.,0.));
#9495=DIRECTION('center_axis',(0.,1.15648231731787E-16,-1.));
#9496=DIRECTION('ref_axis',(0.,1.,1.15648231731787E-16));
#9497=DIRECTION('center_axis',(0.,1.15648231731787E-16,-1.));
#9498=DIRECTION('ref_axis',(0.,1.,1.15648231731787E-16));
#9499=DIRECTION('center_axis',(0.999938130553997,0.,0.0111236263950905));
#9500=DIRECTION('ref_axis',(0.0111236263950905,0.,-0.999938130553997));
#9501=DIRECTION('',(-1.28650731853232E-18,1.,1.15648231731787E-16));
#9502=DIRECTION('center_axis',(0.,0.,1.));
#9503=DIRECTION('ref_axis',(1.,0.,0.));
#9504=DIRECTION('',(-1.,0.,0.));
#9505=DIRECTION('center_axis',(0.,-1.,0.));
#9506=DIRECTION('ref_axis',(-0.0859974399428422,0.,0.996295357975373));
#9507=DIRECTION('',(0.,1.,0.));
#9508=DIRECTION('center_axis',(0.,1.,1.24352412568707E-16));
#9509=DIRECTION('ref_axis',(0.,-1.24352412568707E-16,1.));
#9510=DIRECTION('center_axis',(0.,-1.,-1.24352412568707E-16));
#9511=DIRECTION('ref_axis',(0.,1.24352412568707E-16,-1.));
#9512=DIRECTION('center_axis',(0.,1.,1.24352412568707E-16));
#9513=DIRECTION('ref_axis',(0.,-1.24352412568707E-16,1.));
#9514=DIRECTION('',(0.,1.24352412568707E-16,-1.));
#9515=DIRECTION('',(-1.,0.,0.));
#9516=DIRECTION('center_axis',(0.,-1.,-1.24352412568707E-16));
#9517=DIRECTION('ref_axis',(0.,1.24352412568707E-16,-1.));
#9518=DIRECTION('',(-1.,0.,0.));
#9519=DIRECTION('',(0.,-1.24352412568707E-16,1.));
#9520=DIRECTION('center_axis',(0.,1.15648231731787E-16,-1.));
#9521=DIRECTION('ref_axis',(0.,1.,1.15648231731787E-16));
#9522=DIRECTION('',(0.,-1.,-1.15648231731787E-16));
#9523=DIRECTION('center_axis',(-1.,0.,0.));
#9524=DIRECTION('ref_axis',(0.,0.,1.));
#9525=DIRECTION('center_axis',(1.,0.,-7.88510670898549E-17));
#9526=DIRECTION('ref_axis',(-7.88510670898549E-17,0.,-1.));
#9527=DIRECTION('',(-7.88510670898549E-17,0.,-1.));
#9528=DIRECTION('',(-7.88510670898549E-17,0.,-1.));
#9529=DIRECTION('',(0.,1.,0.));
#9530=DIRECTION('center_axis',(0.,0.,1.));
#9531=DIRECTION('ref_axis',(1.,0.,0.));
#9532=DIRECTION('',(1.,0.,0.));
#9533=DIRECTION('',(0.,1.,0.));
#9534=DIRECTION('',(1.,0.,0.));
#9535=DIRECTION('center_axis',(-1.,0.,1.18276600634782E-16));
#9536=DIRECTION('ref_axis',(1.18276600634782E-16,0.,1.));
#9537=DIRECTION('',(1.18276600634782E-16,0.,1.));
#9538=DIRECTION('',(1.18276600634782E-16,0.,1.));
#9539=DIRECTION('center_axis',(0.,1.,0.));
#9540=DIRECTION('ref_axis',(0.,0.,1.));
#9541=DIRECTION('center_axis',(0.,1.,0.));
#9542=DIRECTION('ref_axis',(0.,0.,1.));
#12301=CARTESIAN_POINT('',(0.,0.,0.));
#12302=CARTESIAN_POINT('Origin',(0.095196568285859,-18.,33.232185266773));
#12303=CARTESIAN_POINT('',(0.0951965682858588,-7.5,31.732185266773));
#12304=CARTESIAN_POINT('Origin',(0.095196568285859,-7.5,33.232185266773));
#12305=CARTESIAN_POINT('',(0.0951965682858588,7.5,31.732185266773));
#12306=CARTESIAN_POINT('',(0.0951965682858588,-18.,31.732185266773));
#12307=CARTESIAN_POINT('Origin',(0.095196568285859,7.5,33.232185266773));
#12308=CARTESIAN_POINT('Origin',(0.0951965682858563,19.8000040922037,8.14863870441721));
#12309=CARTESIAN_POINT('',(0.0951965682858561,-8.24999590779632,9.79863870441721));
#12310=CARTESIAN_POINT('Origin',(0.0951965682858563,-8.24999590779632,8.14863870441721));
#12311=CARTESIAN_POINT('',(0.0951965682858558,-14.0999162292878,9.79863870441721));
#12312=CARTESIAN_POINT('',(0.0951965682858561,19.8000040922037,9.79863870441721));
#12313=CARTESIAN_POINT('',(0.0951965682858563,-14.1575179435509,6.49863870441721));
#12314=CARTESIAN_POINT('Ctrl Pts',(0.0951965682858559,-14.0999162292878,
9.79863870441721));
#12315=CARTESIAN_POINT('Ctrl Pts',(-0.111884389331936,-14.0999162292878,
9.79863870441721));
#12316=CARTESIAN_POINT('Ctrl Pts',(-0.332690322215915,-14.0956093061338,
9.7572743886747));
#12317=CARTESIAN_POINT('Ctrl Pts',(-0.738813012790702,-14.0803572376207,
9.58920247165813));
#12318=CARTESIAN_POINT('Ctrl Pts',(-0.9241426028172,-14.0696692652477,9.46250263892422));
#12319=CARTESIAN_POINT('Ctrl Pts',(-1.21685503126047,-14.0505183636864,
9.17028693794665));
#12320=CARTESIAN_POINT('Ctrl Pts',(-1.34384871039232,-14.0408156535701,
8.98524545523767));
#12321=CARTESIAN_POINT('Ctrl Pts',(-1.5126138598668,-14.0296199070515,8.57957694362764));
#12322=CARTESIAN_POINT('Ctrl Pts',(-1.55437816863629,-14.0283939252263,
8.35893960919315));
#12323=CARTESIAN_POINT('Ctrl Pts',(-1.55522352628415,-14.0355830590593,
7.94423675389232));
#12324=CARTESIAN_POINT('Ctrl Pts',(-1.51404500481727,-14.0445114051257,
7.72278149953618));
#12325=CARTESIAN_POINT('Ctrl Pts',(-1.34599446823065,-14.0698943839908,
7.31558332529204));
#12326=CARTESIAN_POINT('Ctrl Pts',(-1.21913545885449,-14.0860803724786,
7.12981833652177));
#12327=CARTESIAN_POINT('Ctrl Pts',(-0.926341065508513,-14.1154701420388,
6.83642648344605));
#12328=CARTESIAN_POINT('Ctrl Pts',(-0.740831328663387,-14.1305991784691,
6.70916694867708));
#12329=CARTESIAN_POINT('Ctrl Pts',(-0.33394200376843,-14.1517518463386,
6.54026633590998));
#12330=CARTESIAN_POINT('Ctrl Pts',(-0.112543486877898,-14.1575179435509,
6.49863870441721));
#12331=CARTESIAN_POINT('Ctrl Pts',(0.0951965682858563,-14.1575179435509,
6.49863870441721));
#12332=CARTESIAN_POINT('Ctrl Pts',(0.0951965682858563,-14.1575179435509,
6.49863870441721));
#12333=CARTESIAN_POINT('Ctrl Pts',(0.302936623449611,-14.1575179435509,
6.49863870441721));
#12334=CARTESIAN_POINT('Ctrl Pts',(0.524335140340142,-14.1517518463386,
6.54026633590998));
#12335=CARTESIAN_POINT('Ctrl Pts',(0.931224465235098,-14.1305991784691,
6.70916694867708));
#12336=CARTESIAN_POINT('Ctrl Pts',(1.11673420208023,-14.1154701420388,6.83642648344605));
#12337=CARTESIAN_POINT('Ctrl Pts',(1.4095285954262,-14.0860803724786,7.12981833652177));
#12338=CARTESIAN_POINT('Ctrl Pts',(1.53638760480237,-14.0698943839908,7.31558332529205));
#12339=CARTESIAN_POINT('Ctrl Pts',(1.70443814138898,-14.0445114051257,7.72278149953618));
#12340=CARTESIAN_POINT('Ctrl Pts',(1.74561666285586,-14.0355830590593,7.94423675389232));
#12341=CARTESIAN_POINT('Ctrl Pts',(1.74519314013823,-14.0319813154587,8.15200216623844));
#12342=CARTESIAN_POINT('Ctrl Pts',(1.744771305208,-14.0283939252263,8.35893960919316));
#12343=CARTESIAN_POINT('Ctrl Pts',(1.70300699643852,-14.0296199070515,8.57957694362764));
#12344=CARTESIAN_POINT('Ctrl Pts',(1.53424184696403,-14.0408156535701,8.98524545523767));
#12345=CARTESIAN_POINT('Ctrl Pts',(1.40724816783219,-14.0505183636864,9.17028693794665));
#12346=CARTESIAN_POINT('Ctrl Pts',(1.11453573938891,-14.0696692652477,9.46250263892422));
#12347=CARTESIAN_POINT('Ctrl Pts',(0.929206149362414,-14.0803572376207,
9.58920247165813));
#12348=CARTESIAN_POINT('Ctrl Pts',(0.523083458787627,-14.0956093061338,
9.7572743886747));
#12349=CARTESIAN_POINT('Ctrl Pts',(0.302277525903648,-14.0999162292878,
9.79863870441721));
#12350=CARTESIAN_POINT('Ctrl Pts',(0.095196568285856,-14.0999162292878,
9.79863870441721));
#12351=CARTESIAN_POINT('Origin',(0.0951965682858563,19.8000040922037,8.14863870441721));
#12352=CARTESIAN_POINT('',(0.0951965682865928,14.1575261279592,6.49863870441022));
#12353=CARTESIAN_POINT('',(0.0951965682858563,14.0999244136952,9.79863870441721));
#12354=CARTESIAN_POINT('Ctrl Pts',(0.0951965682858558,14.1575261279583,
6.49863870441721));
#12355=CARTESIAN_POINT('Ctrl Pts',(-0.112543486877899,14.1575261279583,
6.49863870441721));
#12356=CARTESIAN_POINT('Ctrl Pts',(-0.33394200376843,14.151760030746,6.54026633590998));
#12357=CARTESIAN_POINT('Ctrl Pts',(-0.740831328663387,14.1306073628765,
6.70916694867708));
#12358=CARTESIAN_POINT('Ctrl Pts',(-0.926341065508513,14.1154783264462,
6.83642648344605));
#12359=CARTESIAN_POINT('Ctrl Pts',(-1.21913545885449,14.0860885568859,7.12981833652177));
#12360=CARTESIAN_POINT('Ctrl Pts',(-1.34599446823065,14.0699025683982,7.31558332529205));
#12361=CARTESIAN_POINT('Ctrl Pts',(-1.51404500481727,14.0445195895331,7.72278149953618));
#12362=CARTESIAN_POINT('Ctrl Pts',(-1.55522352628415,14.0355912434667,7.94423675389232));
#12363=CARTESIAN_POINT('Ctrl Pts',(-1.55437816863629,14.0284021096337,8.35893960919315));
#12364=CARTESIAN_POINT('Ctrl Pts',(-1.5126138598668,14.0296280914589,8.57957694362764));
#12365=CARTESIAN_POINT('Ctrl Pts',(-1.34384871039232,14.0408238379775,8.98524545523767));
#12366=CARTESIAN_POINT('Ctrl Pts',(-1.21685503126047,14.0505265480937,9.17028693794665));
#12367=CARTESIAN_POINT('Ctrl Pts',(-0.9241426028172,14.0696774496551,9.46250263892422));
#12368=CARTESIAN_POINT('Ctrl Pts',(-0.738813012790702,14.080365422028,9.58920247165813));
#12369=CARTESIAN_POINT('Ctrl Pts',(-0.332690322215915,14.0956174905411,
9.7572743886747));
#12370=CARTESIAN_POINT('Ctrl Pts',(-0.111884389331936,14.0999244136952,
9.79863870441721));
#12371=CARTESIAN_POINT('Ctrl Pts',(0.0951965682858565,14.0999244136952,
9.79863870441721));
#12372=CARTESIAN_POINT('',(0.0951965682858561,8.25000409220368,9.79863870441721));
#12373=CARTESIAN_POINT('',(0.0951965682858561,19.8000040922037,9.79863870441721));
#12374=CARTESIAN_POINT('Origin',(0.0951965682858563,8.25000409220368,8.14863870441721));
#12375=CARTESIAN_POINT('Ctrl Pts',(0.0951965682858564,14.0999244136952,
9.79863870441721));
#12376=CARTESIAN_POINT('Ctrl Pts',(0.302277525903648,14.0999244136952,9.79863870441721));
#12377=CARTESIAN_POINT('Ctrl Pts',(0.523083458787627,14.0956174905411,9.7572743886747));
#12378=CARTESIAN_POINT('Ctrl Pts',(0.929206149362414,14.080365422028,9.58920247165813));
#12379=CARTESIAN_POINT('Ctrl Pts',(1.11453573938891,14.0696774496551,9.46250263892422));
#12380=CARTESIAN_POINT('Ctrl Pts',(1.40724816783219,14.0505265480937,9.17028693794665));
#12381=CARTESIAN_POINT('Ctrl Pts',(1.53424184696403,14.0408238379775,8.98524545523767));
#12382=CARTESIAN_POINT('Ctrl Pts',(1.70300699643852,14.0296280914589,8.57957694362764));
#12383=CARTESIAN_POINT('Ctrl Pts',(1.744771305208,14.0284021096337,8.35893960919316));
#12384=CARTESIAN_POINT('Ctrl Pts',(1.74519314013823,14.0319894998661,8.15200216623844));
#12385=CARTESIAN_POINT('Ctrl Pts',(1.74561666285586,14.0355912434667,7.94423675389232));
#12386=CARTESIAN_POINT('Ctrl Pts',(1.70443814138898,14.0445195895331,7.72278149953618));
#12387=CARTESIAN_POINT('Ctrl Pts',(1.53638760480237,14.0699025683982,7.31558332529205));
#12388=CARTESIAN_POINT('Ctrl Pts',(1.4095285954262,14.0860885568859,7.12981833652177));
#12389=CARTESIAN_POINT('Ctrl Pts',(1.11673420208023,14.1154783264462,6.83642648344605));
#12390=CARTESIAN_POINT('Ctrl Pts',(0.931224465235098,14.1306073628765,6.70916694867708));
#12391=CARTESIAN_POINT('Ctrl Pts',(0.524335140340142,14.151760030746,6.54026633590998));
#12392=CARTESIAN_POINT('Ctrl Pts',(0.302936623449611,14.1575261279583,6.49863870441721));
#12393=CARTESIAN_POINT('Ctrl Pts',(0.0951965682858559,14.1575261279583,
6.49863870441721));
#12394=CARTESIAN_POINT('Origin',(0.0951965682858563,4.09220368528653E-6,
25.8360815995708));
#12395=CARTESIAN_POINT('',(1.85391052501785,-13.7076189828105,25.8360815995708));
#12396=CARTESIAN_POINT('',(1.85391052501785,-7.5,25.8360815995708));
#12397=CARTESIAN_POINT('',(1.85391052501785,20.,25.8360815995708));
#12398=CARTESIAN_POINT('',(-1.66465324600953,-7.5,25.8360815995708));
#12399=CARTESIAN_POINT('',(0.0951965682858563,-7.5,25.8360815995708));
#12400=CARTESIAN_POINT('',(-1.66465324600953,-13.7074732023021,25.8360815995708));
#12401=CARTESIAN_POINT('',(-1.66465324600953,20.,25.8360815995708));
#12402=CARTESIAN_POINT('Origin',(0.0951965682858563,4.09220368528653E-6,
25.8360815995708));
#12403=CARTESIAN_POINT('Origin',(0.0946286395041643,20.,3.93764471879911));
#12404=CARTESIAN_POINT('',(5.09519656828586,-7.5,25.329954808256));
#12405=CARTESIAN_POINT('',(5.09519656828586,7.5,25.329954808256));
#12406=CARTESIAN_POINT('',(5.09519656828586,20.,25.329954808256));
#12407=CARTESIAN_POINT('Origin',(0.0946286395041643,-7.5,3.93764471879911));
#12408=CARTESIAN_POINT('',(13.9148485158407,-1.53043517371412,21.0150605989476));
#12409=CARTESIAN_POINT('Ctrl Pts',(1.85391052501786,-13.7076189828105,25.8360815995708));
#12410=CARTESIAN_POINT('Ctrl Pts',(2.17648767471965,-13.6666877855093,25.8101663189852));
#12411=CARTESIAN_POINT('Ctrl Pts',(2.49904065381574,-13.6142947682306,25.777060184476));
#12412=CARTESIAN_POINT('Ctrl Pts',(3.72754363797017,-13.3699910032897,25.6234687931974));
#12413=CARTESIAN_POINT('Ctrl Pts',(4.62247333626519,-13.0970219827471,25.4529090529867));
#12414=CARTESIAN_POINT('Ctrl Pts',(7.17708557690186,-12.030828714843,24.8077398984456));
#12415=CARTESIAN_POINT('Ctrl Pts',(8.70490101058748,-10.9780802446545,24.1936108601555));
#12416=CARTESIAN_POINT('Ctrl Pts',(11.1212920908085,-8.58574185129343,22.9873702251227));
#12417=CARTESIAN_POINT('Ctrl Pts',(12.1830463956658,-7.06841765762853,22.303147136569));
#12418=CARTESIAN_POINT('Ctrl Pts',(13.2627850426251,-4.53156635476595,21.5283391995247));
#12419=CARTESIAN_POINT('Ctrl Pts',(13.540303942053,-3.64206254291784,21.3130804475981));
#12420=CARTESIAN_POINT('Ctrl Pts',(13.8061400403014,-2.33638296572343,21.1027786503388));
#12421=CARTESIAN_POINT('Ctrl Pts',(13.8695513851653,-1.93364874310124,21.0517181535856));
#12422=CARTESIAN_POINT('Ctrl Pts',(13.9148485158408,-1.53043517371412,21.0150605989476));
#12423=CARTESIAN_POINT('',(13.9148485158407,1.53044335812149,21.0150605989476));
#12424=CARTESIAN_POINT('',(13.9148485158407,20.,21.0150605989476));
#12425=CARTESIAN_POINT('',(1.85391052501785,13.7076271672179,25.8360815995708));
#12426=CARTESIAN_POINT('Ctrl Pts',(13.9148485158408,1.5304433581215,21.0150605989476));
#12427=CARTESIAN_POINT('Ctrl Pts',(13.8695513851653,1.93365692750862,21.0517181535856));
#12428=CARTESIAN_POINT('Ctrl Pts',(13.8061400403014,2.33639115013081,21.1027786503388));
#12429=CARTESIAN_POINT('Ctrl Pts',(13.5403039420529,3.64207072732521,21.3130804475981));
#12430=CARTESIAN_POINT('Ctrl Pts',(13.2627850426251,4.53157453917333,21.5283391995247));
#12431=CARTESIAN_POINT('Ctrl Pts',(12.1830463956658,7.0684258420359,22.303147136569));
#12432=CARTESIAN_POINT('Ctrl Pts',(11.1212920908085,8.58575003570079,22.9873702251227));
#12433=CARTESIAN_POINT('Ctrl Pts',(8.70490101058748,10.9780884290619,24.1936108601555));
#12434=CARTESIAN_POINT('Ctrl Pts',(7.17708557690186,12.0308368992504,24.8077398984456));
#12435=CARTESIAN_POINT('Ctrl Pts',(4.62247333626519,13.0970301671545,25.4529090529867));
#12436=CARTESIAN_POINT('Ctrl Pts',(3.72754363797016,13.3699991876971,25.6234687931974));
#12437=CARTESIAN_POINT('Ctrl Pts',(2.49904065381574,13.6143029526379,25.777060184476));
#12438=CARTESIAN_POINT('Ctrl Pts',(2.17648767471964,13.6666959699166,25.8101663189852));
#12439=CARTESIAN_POINT('Ctrl Pts',(1.85391052501785,13.7076271672179,25.8360815995708));
#12440=CARTESIAN_POINT('',(1.85391052501785,7.5,25.8360815995708));
#12441=CARTESIAN_POINT('',(1.85391052501785,20.,25.8360815995708));
#12442=CARTESIAN_POINT('Origin',(0.0946286395041643,7.5,3.93764471879911));
#12443=CARTESIAN_POINT('Origin',(0.0946286395041643,20.,3.93764471879911));
#12444=CARTESIAN_POINT('',(-4.90480343171414,-7.5,25.3302202892888));
#12445=CARTESIAN_POINT('Origin',(0.0946286395041643,-7.5,3.93764471879911));
#12446=CARTESIAN_POINT('',(-4.90480343171414,7.5,25.3302202892888));
#12447=CARTESIAN_POINT('',(-4.90480343171414,20.,25.3302202892888));
#12448=CARTESIAN_POINT('',(-1.66465324600953,7.5,25.8360815995708));
#12449=CARTESIAN_POINT('Origin',(0.0946286395041643,7.5,3.93764471879911));
#12450=CARTESIAN_POINT('',(-1.66465324600953,13.7074813867094,25.8360815995708));
#12451=CARTESIAN_POINT('',(-1.66465324600953,20.,25.8360815995708));
#12452=CARTESIAN_POINT('Ctrl Pts',(-1.66465324600953,13.7074813867094,25.8360815995708));
#12453=CARTESIAN_POINT('Ctrl Pts',(-1.98684074890723,13.666572498391,25.8101976225238));
#12454=CARTESIAN_POINT('Ctrl Pts',(-2.30900267606637,13.6142293374932,25.7771403165208));
#12455=CARTESIAN_POINT('Ctrl Pts',(-3.53711118769133,13.3700057780211,25.6236650528541));
#12456=CARTESIAN_POINT('Ctrl Pts',(-4.43203636345268,13.0970405100357,25.4531566824588));
#12457=CARTESIAN_POINT('Ctrl Pts',(-6.98664158061922,12.0308577278043,24.8081401060509));
#12458=CARTESIAN_POINT('Ctrl Pts',(-8.51446121511986,10.9781143124401,24.1941111489798));
#12459=CARTESIAN_POINT('Ctrl Pts',(-10.9308714321239,8.58576963670896,22.9880418512269));
#12460=CARTESIAN_POINT('Ctrl Pts',(-11.9926351420235,7.06843317708346,22.3039048439548));
#12461=CARTESIAN_POINT('Ctrl Pts',(-13.0723782208733,4.53156918261022,21.5291992027477));
#12462=CARTESIAN_POINT('Ctrl Pts',(-13.3498970434732,3.64206232315039,21.3139698195036));
#12463=CARTESIAN_POINT('Ctrl Pts',(-13.7188857908144,1.82973119863964,21.0221044535754));
#12464=CARTESIAN_POINT('Ctrl Pts',(-13.8101407844913,0.90673105293582,20.9462895160591));
#12465=CARTESIAN_POINT('Ctrl Pts',(-13.8101407844913,-0.906722868528451,
20.9462895160591));
#12466=CARTESIAN_POINT('Ctrl Pts',(-13.7188857908144,-1.82972301423227,
21.0221044535754));
#12467=CARTESIAN_POINT('Ctrl Pts',(-13.3498970434732,-3.64205413874302,
21.3139698195036));
#12468=CARTESIAN_POINT('Ctrl Pts',(-13.0723782208733,-4.53156099820285,
21.5291992027477));
#12469=CARTESIAN_POINT('Ctrl Pts',(-11.9926351420235,-7.06842499267609,
22.3039048439548));
#12470=CARTESIAN_POINT('Ctrl Pts',(-10.9308714321239,-8.58576145230159,
22.9880418512269));
#12471=CARTESIAN_POINT('Ctrl Pts',(-8.51446121511986,-10.9781061280328,
24.1941111489798));
#12472=CARTESIAN_POINT('Ctrl Pts',(-6.98664158061922,-12.0308495433969,
24.8081401060509));
#12473=CARTESIAN_POINT('Ctrl Pts',(-4.43203636345268,-13.0970323256283,
25.4531566824588));
#12474=CARTESIAN_POINT('Ctrl Pts',(-3.53711118769134,-13.3699975936137,
25.6236650528541));
#12475=CARTESIAN_POINT('Ctrl Pts',(-2.30900267606638,-13.6142211530858,
25.7771403165208));
#12476=CARTESIAN_POINT('Ctrl Pts',(-1.98684074890723,-13.6665643139837,
25.8101976225238));
#12477=CARTESIAN_POINT('Ctrl Pts',(-1.66465324600953,-13.7074732023021,
25.8360815995708));
#12478=CARTESIAN_POINT('Origin',(0.0951965682858563,4.09220368528653E-6,
-1.66391840042922));
#12479=CARTESIAN_POINT('Origin',(0.0951965682858563,4.09220368528653E-6,
25.8360815995708));
#12480=CARTESIAN_POINT('',(13.9964332854894,1.91230024237248,13.6811463567195));
#12481=CARTESIAN_POINT('Ctrl Pts',(13.9964332854889,1.91230024237026,13.6811463567665));
#12482=CARTESIAN_POINT('Ctrl Pts',(13.9511163435649,1.71995846239176,17.7548302958379));
#12483=CARTESIAN_POINT('Ctrl Pts',(13.9148485158408,1.53044335812149,21.0150605989476));
#12484=CARTESIAN_POINT('',(11.4459127938674,8.25000409220368,13.6811463567195));
#12485=CARTESIAN_POINT('Origin',(0.0951965682858563,4.0922036817656E-6,
13.6811463567195));
#12486=CARTESIAN_POINT('',(11.7275471444307,8.25000409220369,0.574489862137293));
#12487=CARTESIAN_POINT('Ctrl Pts',(11.7275471444307,8.25000409220369,0.574489862137293));
#12488=CARTESIAN_POINT('Ctrl Pts',(11.7222207733811,8.25000409220369,0.823392575266454));
#12489=CARTESIAN_POINT('Ctrl Pts',(11.7168931785629,8.25000409220369,1.07229526221072));
#12490=CARTESIAN_POINT('Ctrl Pts',(11.7115643549194,8.25000409220369,1.32119792284374));
#12491=CARTESIAN_POINT('Ctrl Pts',(11.623358382574,8.25000409220369,5.4411881250697));
#12492=CARTESIAN_POINT('Ctrl Pts',(11.5348159240829,8.25000409220368,9.5611711391444));
#12493=CARTESIAN_POINT('Ctrl Pts',(11.4459127938674,8.25000409220368,13.6811463567195));
#12494=CARTESIAN_POINT('',(11.7275471444307,-8.24999590779632,0.574489862137297));
#12495=CARTESIAN_POINT('Ctrl Pts',(11.7275471444307,-8.24999590779632,0.574489862137297));
#12496=CARTESIAN_POINT('Ctrl Pts',(11.2506528785961,-8.91132535705997,0.941801995911842));
#12497=CARTESIAN_POINT('Ctrl Pts',(10.7233874704347,-9.52161727744828,1.31121249637851));
#12498=CARTESIAN_POINT('Ctrl Pts',(8.94944501462999,-11.2682573787269,2.41723416442409));
#12499=CARTESIAN_POINT('Ctrl Pts',(7.39695628067307,-12.3428102097436,3.18167544610478));
#12500=CARTESIAN_POINT('Ctrl Pts',(4.77843360940769,-13.4402628572067,3.98877045439691));
#12501=CARTESIAN_POINT('Ctrl Pts',(3.85772926770378,-13.723285699755,4.20321806216009));
#12502=CARTESIAN_POINT('Ctrl Pts',(1.98310564117687,-14.0988472144289,4.49284734361978));
#12503=CARTESIAN_POINT('Ctrl Pts',(1.02913009218085,-14.1912194513045,4.56788061831652));
#12504=CARTESIAN_POINT('Ctrl Pts',(-0.837205424454879,-14.1910264736106,
4.57893630299566));
#12505=CARTESIAN_POINT('Ctrl Pts',(-1.79050220705526,-14.0987476035694,
4.51541564045522));
#12506=CARTESIAN_POINT('Ctrl Pts',(-3.66513456872354,-13.7230644103538,
4.24895350849291));
#12507=CARTESIAN_POINT('Ctrl Pts',(-4.58652368156226,-13.4398199148439,
4.04616337164375));
#12508=CARTESIAN_POINT('Ctrl Pts',(-7.20822347504013,-12.340360202428,3.27354943135428));
#12509=CARTESIAN_POINT('Ctrl Pts',(-8.7643920193079,-11.2624168750667,2.53153132261272));
#12510=CARTESIAN_POINT('Ctrl Pts',(-11.2319892354444,-8.8269552131712,1.03862052793401));
#12511=CARTESIAN_POINT('Ctrl Pts',(-12.317306699732,-7.28274628710442,0.167204139697448));
#12512=CARTESIAN_POINT('Ctrl Pts',(-13.4306122032903,-4.6928986142151,-0.858100732123217));
#12513=CARTESIAN_POINT('Ctrl Pts',(-13.7190471318454,-3.78298207865309,
-1.15053717027747));
#12514=CARTESIAN_POINT('Ctrl Pts',(-14.1062637700055,-1.91424092738689,
-1.55431913138643));
#12515=CARTESIAN_POINT('Ctrl Pts',(-14.2048034317141,-0.954989281852873,
-1.66391840042921));
#12516=CARTESIAN_POINT('Ctrl Pts',(-14.2048034317141,0.954997466260247,
-1.66391840042921));
#12517=CARTESIAN_POINT('Ctrl Pts',(-14.1062637700055,1.91424911179426,-1.55431913138642));
#12518=CARTESIAN_POINT('Ctrl Pts',(-13.7190471318454,3.78299026306046,-1.15053717027747));
#12519=CARTESIAN_POINT('Ctrl Pts',(-13.4306122032903,4.69290679862247,-0.85810073212322));
#12520=CARTESIAN_POINT('Ctrl Pts',(-12.317306699732,7.28275447151178,0.167204139697442));
#12521=CARTESIAN_POINT('Ctrl Pts',(-11.2319892354444,8.82696339757856,1.03862052793401));
#12522=CARTESIAN_POINT('Ctrl Pts',(-8.7643920193079,11.2624250594741,2.53153132261272));
#12523=CARTESIAN_POINT('Ctrl Pts',(-7.20822347504013,12.3403683868354,3.27354943135428));
#12524=CARTESIAN_POINT('Ctrl Pts',(-4.58652368156226,13.4398280992513,4.04616337164375));
#12525=CARTESIAN_POINT('Ctrl Pts',(-3.66513456872355,13.7230725947612,4.24895350849291));
#12526=CARTESIAN_POINT('Ctrl Pts',(-1.79050220705526,14.0987557879767,4.51541564045522));
#12527=CARTESIAN_POINT('Ctrl Pts',(-0.837205424454882,14.191034658018,4.57893630299566));
#12528=CARTESIAN_POINT('Ctrl Pts',(1.03171319044408,14.1912279028023,4.56786531671633));
#12529=CARTESIAN_POINT('Ctrl Pts',(1.98817223795939,14.0983467992742,4.49243379841232));
#12530=CARTESIAN_POINT('Ctrl Pts',(3.86732265571208,13.720861540725,4.2013637484486));
#12531=CARTESIAN_POINT('Ctrl Pts',(4.79007085667628,13.4364250401153,3.98587473350674));
#12532=CARTESIAN_POINT('Ctrl Pts',(7.41380568479443,12.3336701876795,3.1750837142893));
#12533=CARTESIAN_POINT('Ctrl Pts',(8.96853555697387,11.2541395041803,2.40738046212495));
#12534=CARTESIAN_POINT('Ctrl Pts',(10.7357556493519,9.50728123601757,1.3025507908185));
#12535=CARTESIAN_POINT('Ctrl Pts',(11.256192956559,8.90365088103174,0.937534932951304));
#12536=CARTESIAN_POINT('Ctrl Pts',(11.7275471444307,8.25000409220369,0.574489862137297));
#12537=CARTESIAN_POINT('',(11.4459127938674,-8.24999590779632,13.6811463567195));
#12538=CARTESIAN_POINT('Ctrl Pts',(11.4459127938674,-8.24999590779632,13.6811463567195));
#12539=CARTESIAN_POINT('Ctrl Pts',(11.5348159240829,-8.24999590779632,9.56117113914441));
#12540=CARTESIAN_POINT('Ctrl Pts',(11.623358382574,-8.24999590779632,5.44118812506971));
#12541=CARTESIAN_POINT('Ctrl Pts',(11.7115643549194,-8.24999590779632,1.32119792284375));
#12542=CARTESIAN_POINT('Ctrl Pts',(11.7168931785629,-8.24999590779632,1.07229526221074));
#12543=CARTESIAN_POINT('Ctrl Pts',(11.7222207733811,-8.24999590779632,0.823392575266463));
#12544=CARTESIAN_POINT('Ctrl Pts',(11.7275471444307,-8.24999590779632,0.574489862137297));
#12545=CARTESIAN_POINT('',(13.9964332854894,-1.9122920579651,13.6811463567195));
#12546=CARTESIAN_POINT('Origin',(0.0951965682858563,4.0922036817656E-6,
13.6811463567195));
#12547=CARTESIAN_POINT('Ctrl Pts',(13.9148485158427,-1.53043517372403,21.015060598777));
#12548=CARTESIAN_POINT('Ctrl Pts',(13.9511163435661,-1.71995027798942,17.7548302957312));
#12549=CARTESIAN_POINT('Ctrl Pts',(13.9964332854889,-1.91229205796288,13.6811463567667));
#12550=CARTESIAN_POINT('Origin',(14.1653954217721,39.6000040922037,-1.5073970811911));
#12551=CARTESIAN_POINT('',(13.9964332854894,39.6000040922037,13.6811463567195));
#12552=CARTESIAN_POINT('Origin',(0.0951965682858563,4.09220368528653E-6,
25.8360815995708));
#12553=CARTESIAN_POINT('',(0.0951965682858563,7.5,25.8360815995708));
#12554=CARTESIAN_POINT('Origin',(-0.0188334087686722,39.6000040922037,-14.6762492641943));
#12555=CARTESIAN_POINT('',(-8.70480343171414,-8.24999590779632,2.50270369460076));
#12556=CARTESIAN_POINT('',(-8.70480343171414,8.25000409220368,2.50270369460076));
#12557=CARTESIAN_POINT('',(-8.70480343171414,39.6000040922037,2.50270369460077));
#12558=CARTESIAN_POINT('Origin',(-0.0188334087686722,-8.24999590779631,
-14.6762492641943));
#12559=CARTESIAN_POINT('Origin',(-0.0188334087686722,8.25000409220369,-14.6762492641943));
#12560=CARTESIAN_POINT('Origin',(17.6951965682859,-8.24999590779631,-17.008983157578));
#12561=CARTESIAN_POINT('',(-8.70480343171414,-8.24999590779632,13.6811463567195));
#12562=CARTESIAN_POINT('',(-8.70480343171414,-8.24999590779631,-17.008983157578));
#12563=CARTESIAN_POINT('',(17.6951965682859,-8.24999590779632,13.6811463567195));
#12564=CARTESIAN_POINT('Origin',(17.6951965682859,8.25000409220369,-17.0089831575779));
#12565=CARTESIAN_POINT('',(-8.70480343171414,8.25000409220368,13.6811463567195));
#12566=CARTESIAN_POINT('',(17.6951965682859,8.25000409220368,13.6811463567195));
#12567=CARTESIAN_POINT('',(-8.70480343171414,8.25000409220369,-17.0089831575779));
#12568=CARTESIAN_POINT('Origin',(17.6951965682859,8.25000409220368,13.6811463567195));
#12569=CARTESIAN_POINT('',(-8.70480343171414,8.25000409220368,13.6811463567195));
#12570=CARTESIAN_POINT('Origin',(-8.70480343171414,4.09220368528653E-6,
-1.66391840042922));
#12571=CARTESIAN_POINT('Origin',(5.09519656828586,-7.5,14.732185266773));
#12572=CARTESIAN_POINT('',(5.09519656828586,-7.5,36.732185266773));
#12573=CARTESIAN_POINT('',(5.09519656828586,-7.5,14.732185266773));
#12574=CARTESIAN_POINT('',(5.09519656828586,7.5,36.732185266773));
#12575=CARTESIAN_POINT('',(5.09519656828586,7.5,14.732185266773));
#12576=CARTESIAN_POINT('',(5.09519656828586,-7.5,36.732185266773));
#12577=CARTESIAN_POINT('Origin',(-4.90480343171414,-7.5,36.732185266773));
#12578=CARTESIAN_POINT('',(-4.90480343171414,7.5,36.732185266773));
#12579=CARTESIAN_POINT('',(-4.90480343171414,7.5,36.732185266773));
#12580=CARTESIAN_POINT('',(-4.90480343171414,-7.5,36.732185266773));
#12581=CARTESIAN_POINT('',(-4.90480343171414,-7.5,36.732185266773));
#12582=CARTESIAN_POINT('',(-4.90480343171414,-7.5,36.732185266773));
#12583=CARTESIAN_POINT('Origin',(-4.90480343171414,-7.5,14.732185266773));
#12584=CARTESIAN_POINT('',(-4.90480343171414,7.5,14.732185266773));
#12585=CARTESIAN_POINT('',(-4.90480343171414,-7.5,14.732185266773));
#12586=CARTESIAN_POINT('Origin',(0.,-7.5,0.));
#12587=CARTESIAN_POINT('Origin',(0.,7.5,0.));
#13167=UNCERTAINTY_MEASURE_WITH_UNIT(LENGTH_MEASURE(0.01),#13200,
'DISTANCE_ACCURACY_VALUE',
'Maximum model space distance between geometric entities at asserted c
onnectivities');
#13173=UNCERTAINTY_MEASURE_WITH_UNIT(LENGTH_MEASURE(0.01),#13200,
'DISTANCE_ACCURACY_VALUE',
'Maximum model space distance between geometric entities at asserted c
onnectivities');
#13193=(
GEOMETRIC_REPRESENTATION_CONTEXT(3)
GLOBAL_UNCERTAINTY_ASSIGNED_CONTEXT((#13167))
GLOBAL_UNIT_ASSIGNED_CONTEXT((#13200,#13202,#13203))
REPRESENTATION_CONTEXT('','3D')
);
#13199=(
GEOMETRIC_REPRESENTATION_CONTEXT(3)
GLOBAL_UNCERTAINTY_ASSIGNED_CONTEXT((#13173))
GLOBAL_UNIT_ASSIGNED_CONTEXT((#13200,#13202,#13203))
REPRESENTATION_CONTEXT('','3D')
);
#13200=(
LENGTH_UNIT()
NAMED_UNIT(*)
SI_UNIT(.MILLI.,.METRE.)
);
#13202=(
NAMED_UNIT(*)
PLANE_ANGLE_UNIT()
SI_UNIT($,.RADIAN.)
);
#13203=(
NAMED_UNIT(*)
SI_UNIT($,.STERADIAN.)
SOLID_ANGLE_UNIT()
);
#13223=SHAPE_DEFINITION_REPRESENTATION(#13262,#13297);
#13262=PRODUCT_DEFINITION_SHAPE('',$,#13323);
#13297=SHAPE_REPRESENTATION('',(#7666),#13193);
#13303=PRODUCT_DEFINITION_CONTEXT('part definition',#13380,'design');
#13323=PRODUCT_DEFINITION('Thumb Link 1','Thumb Link 1',#13348,#13303);
#13348=PRODUCT_DEFINITION_FORMATION('',$,#13401);
#13380=APPLICATION_CONTEXT(
'Core Data for Automotive Mechanical Design Process');
#13381=PRODUCT_CONTEXT('part definition',#13380,'mechanical');
#13401=PRODUCT('Thumb Link 1','Thumb Link 1',$,(#13381));
#13411=PRESENTATION_STYLE_ASSIGNMENT((#13416));
#13416=SURFACE_STYLE_USAGE(.BOTH.,#13421);
#13421=SURFACE_SIDE_STYLE('',(#13426));
#13426=SURFACE_STYLE_FILL_AREA(#13431);
#13431=FILL_AREA_STYLE('Opaque(97,158,199)',(#13436));
#13436=FILL_AREA_STYLE_COLOUR('Opaque(97,158,199)',#13441);
#13441=COLOUR_RGB('Opaque(97,158,199)',0.380392156862745,0.619607843137255,
0.780392156862745);
ENDSEC;
END-ISO-10303-21;
